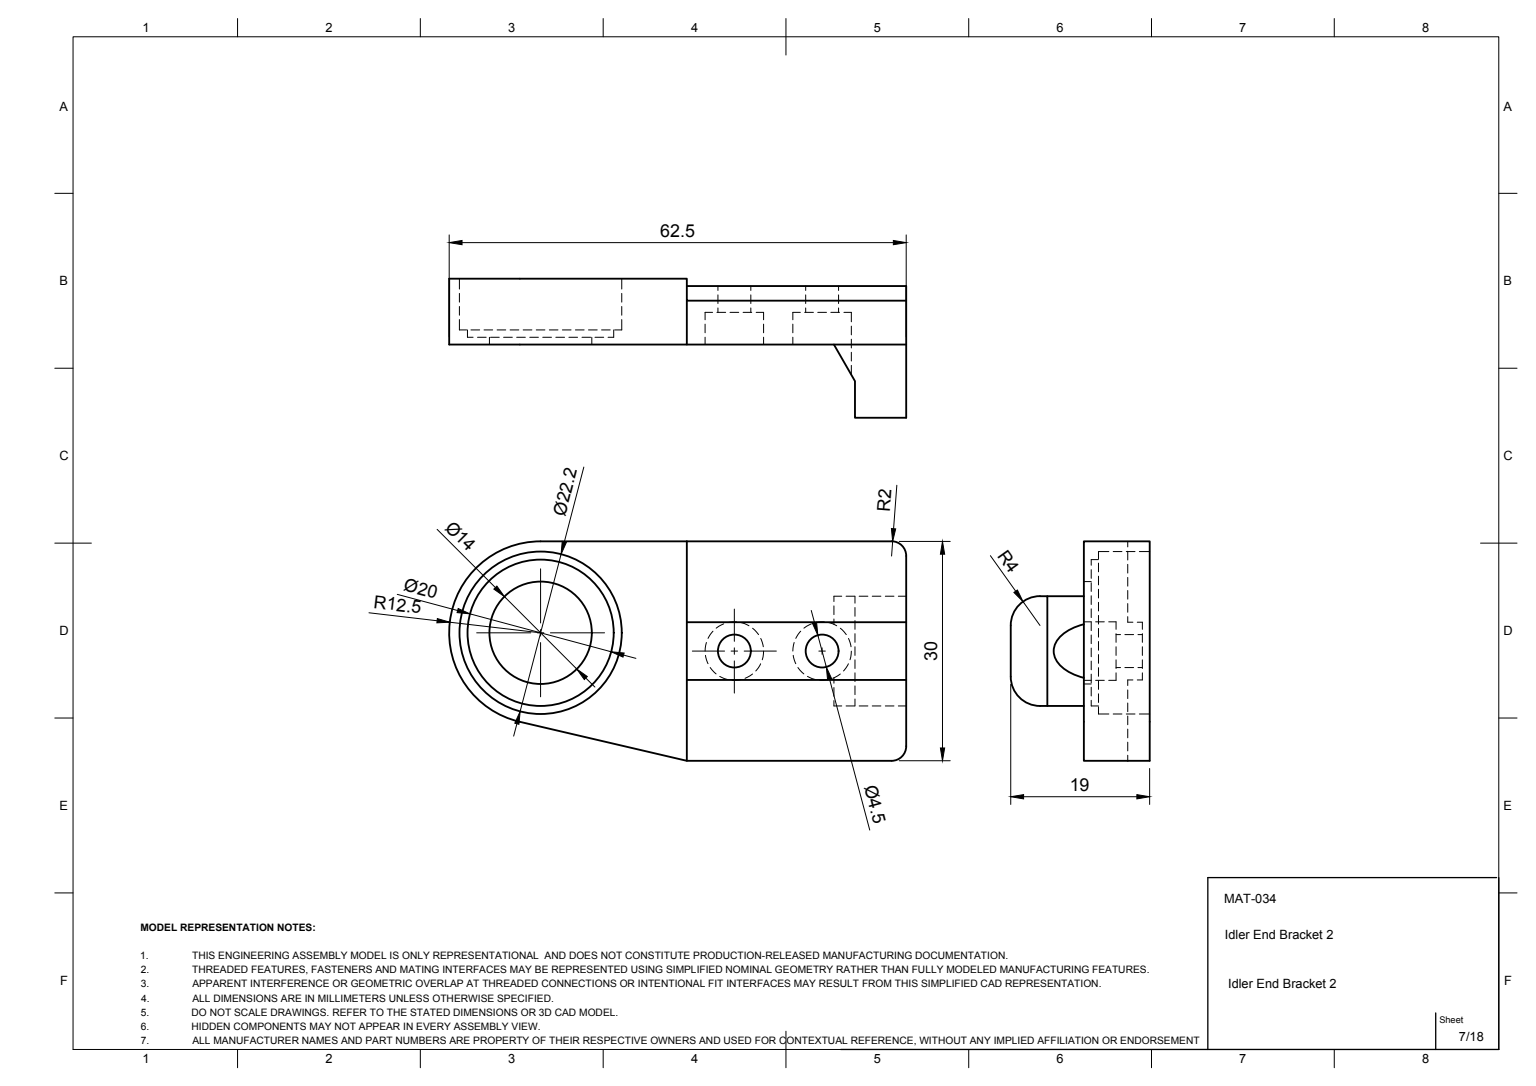
ISO-10303-21;
HEADER;
/* Generated by software containing ST-Developer
 * from STEP Tools, Inc. (www.steptools.com) 
 */

FILE_DESCRIPTION(
/* description */ ('STEP AP214'),
/* implementation_level */ '2;1');

FILE_NAME(
/* name */ 'Idler End Bracket 2.step',
/* time_stamp */ '2026-11-14T09:24:36-08:00',
/* author */ (''),
/* organization */ (''),
/* preprocessor_version */ 'ST-DEVELOPER v20.2',
/* originating_system */ 'Autodesk Translation Framework v15.17.0.0',
/* authorisation */ '');

FILE_SCHEMA (('AUTOMOTIVE_DESIGN { 1 0 10303 214 3 1 1 }'));
ENDSEC;

DATA;
#10=MECHANICAL_DESIGN_GEOMETRIC_PRESENTATION_REPRESENTATION('',(#206),#18867);
#169=ELLIPSE('',#11369,7.99999999999924,3.99999999999989);
#170=ELLIPSE('',#11371,7.99999999999924,3.99999999999989);
#174=SHAPE_REPRESENTATION_RELATIONSHIP('SRR','None',#18938,#190);
#190=ADVANCED_BREP_SHAPE_REPRESENTATION('',(#230),#18854);
#206=STYLED_ITEM('',(#19025),#230);
#230=MANIFOLD_SOLID_BREP('Body1',#10961);
#292=FACE_BOUND('',#1507,.T.);
#293=FACE_BOUND('',#1508,.T.);
#294=FACE_BOUND('',#1510,.T.);
#295=FACE_BOUND('',#1512,.T.);
#296=FACE_BOUND('',#1514,.T.);
#297=FACE_BOUND('',#1518,.T.);
#298=FACE_BOUND('',#1520,.T.);
#299=FACE_BOUND('',#1529,.T.);
#300=FACE_BOUND('',#1530,.T.);
#474=PLANE('',#11390);
#475=PLANE('',#11392);
#476=PLANE('',#11394);
#477=PLANE('',#11395);
#478=PLANE('',#11399);
#479=PLANE('',#11400);
#480=PLANE('',#11403);
#481=PLANE('',#11404);
#482=PLANE('',#11407);
#483=PLANE('',#11408);
#484=PLANE('',#11409);
#485=PLANE('',#11412);
#486=PLANE('',#11413);
#487=PLANE('',#11414);
#488=PLANE('',#11415);
#489=PLANE('',#11418);
#490=PLANE('',#11419);
#491=PLANE('',#11422);
#492=PLANE('',#11423);
#493=PLANE('',#11424);
#494=PLANE('',#11425);
#854=FACE_OUTER_BOUND('',#1491,.T.);
#855=FACE_OUTER_BOUND('',#1492,.T.);
#856=FACE_OUTER_BOUND('',#1493,.T.);
#857=FACE_OUTER_BOUND('',#1494,.T.);
#858=FACE_OUTER_BOUND('',#1495,.T.);
#859=FACE_OUTER_BOUND('',#1496,.T.);
#860=FACE_OUTER_BOUND('',#1497,.T.);
#861=FACE_OUTER_BOUND('',#1498,.T.);
#862=FACE_OUTER_BOUND('',#1499,.T.);
#863=FACE_OUTER_BOUND('',#1500,.T.);
#864=FACE_OUTER_BOUND('',#1501,.T.);
#865=FACE_OUTER_BOUND('',#1502,.T.);
#866=FACE_OUTER_BOUND('',#1503,.T.);
#867=FACE_OUTER_BOUND('',#1504,.T.);
#868=FACE_OUTER_BOUND('',#1505,.T.);
#869=FACE_OUTER_BOUND('',#1506,.T.);
#870=FACE_OUTER_BOUND('',#1509,.T.);
#871=FACE_OUTER_BOUND('',#1511,.T.);
#872=FACE_OUTER_BOUND('',#1513,.T.);
#873=FACE_OUTER_BOUND('',#1515,.T.);
#874=FACE_OUTER_BOUND('',#1516,.T.);
#875=FACE_OUTER_BOUND('',#1517,.T.);
#876=FACE_OUTER_BOUND('',#1519,.T.);
#877=FACE_OUTER_BOUND('',#1521,.T.);
#878=FACE_OUTER_BOUND('',#1522,.T.);
#879=FACE_OUTER_BOUND('',#1523,.T.);
#880=FACE_OUTER_BOUND('',#1524,.T.);
#881=FACE_OUTER_BOUND('',#1525,.T.);
#882=FACE_OUTER_BOUND('',#1526,.T.);
#883=FACE_OUTER_BOUND('',#1527,.T.);
#884=FACE_OUTER_BOUND('',#1528,.T.);
#885=FACE_OUTER_BOUND('',#1531,.T.);
#886=FACE_OUTER_BOUND('',#1532,.T.);
#1491=EDGE_LOOP('',(#7750,#7751,#7752,#7753,#7754,#7755));
#1492=EDGE_LOOP('',(#7756,#7757,#7758,#7759));
#1493=EDGE_LOOP('',(#7760,#7761,#7762,#7763));
#1494=EDGE_LOOP('',(#7764,#7765,#7766,#7767));
#1495=EDGE_LOOP('',(#7768,#7769,#7770,#7771));
#1496=EDGE_LOOP('',(#7772,#7773,#7774,#7775));
#1497=EDGE_LOOP('',(#7776,#7777,#7778,#7779));
#1498=EDGE_LOOP('',(#7780,#7781,#7782,#7783,#7784));
#1499=EDGE_LOOP('',(#7785,#7786,#7787,#7788,#7789));
#1500=EDGE_LOOP('',(#7790,#7791,#7792,#7793,#7794,#7795,#7796,#7797));
#1501=EDGE_LOOP('',(#7798,#7799,#7800,#7801,#7802));
#1502=EDGE_LOOP('',(#7803,#7804,#7805,#7806));
#1503=EDGE_LOOP('',(#7807,#7808,#7809,#7810,#7811,#7812));
#1504=EDGE_LOOP('',(#7813,#7814,#7815,#7816,#7817,#7818,#7819,#7820,#7821,
#7822,#7823,#7824,#7825,#7826));
#1505=EDGE_LOOP('',(#7827,#7828,#7829,#7830));
#1506=EDGE_LOOP('',(#7831,#7832,#7833,#7834,#7835,#7836,#7837,#7838,#7839,
#7840,#7841,#7842,#7843));
#1507=EDGE_LOOP('',(#7844));
#1508=EDGE_LOOP('',(#7845));
#1509=EDGE_LOOP('',(#7846,#7847,#7848,#7849));
#1510=EDGE_LOOP('',(#7850));
#1511=EDGE_LOOP('',(#7851));
#1512=EDGE_LOOP('',(#7852));
#1513=EDGE_LOOP('',(#7853));
#1514=EDGE_LOOP('',(#7854));
#1515=EDGE_LOOP('',(#7855,#7856,#7857,#7858));
#1516=EDGE_LOOP('',(#7859,#7860,#7861,#7862));
#1517=EDGE_LOOP('',(#7863));
#1518=EDGE_LOOP('',(#7864));
#1519=EDGE_LOOP('',(#7865));
#1520=EDGE_LOOP('',(#7866));
#1521=EDGE_LOOP('',(#7867,#7868,#7869,#7870,#7871));
#1522=EDGE_LOOP('',(#7872,#7873,#7874,#7875,#7876,#7877));
#1523=EDGE_LOOP('',(#7878,#7879,#7880,#7881,#7882));
#1524=EDGE_LOOP('',(#7883,#7884,#7885,#7886));
#1525=EDGE_LOOP('',(#7887,#7888,#7889,#7890));
#1526=EDGE_LOOP('',(#7891,#7892,#7893,#7894));
#1527=EDGE_LOOP('',(#7895,#7896,#7897,#7898,#7899,#7900,#7901));
#1528=EDGE_LOOP('',(#7902,#7903,#7904,#7905));
#1529=EDGE_LOOP('',(#7906));
#1530=EDGE_LOOP('',(#7907));
#1531=EDGE_LOOP('',(#7908,#7909,#7910,#7911));
#1532=EDGE_LOOP('',(#7912,#7913,#7914,#7915));
#2294=LINE('',#16277,#3308);
#2295=LINE('',#16287,#3309);
#2296=LINE('',#16293,#3310);
#2297=LINE('',#16299,#3311);
#2298=LINE('',#16305,#3312);
#2299=LINE('',#16311,#3313);
#2300=LINE('',#16317,#3314);
#2301=LINE('',#16322,#3315);
#2302=LINE('',#16324,#3316);
#2303=LINE('',#16328,#3317);
#2304=LINE('',#16329,#3318);
#2305=LINE('',#16333,#3319);
#2306=LINE('',#16335,#3320);
#2307=LINE('',#16337,#3321);
#2308=LINE('',#16340,#3322);
#2309=LINE('',#16343,#3323);
#2310=LINE('',#16345,#3324);
#2311=LINE('',#16347,#3325);
#2312=LINE('',#16348,#3326);
#2313=LINE('',#16350,#3327);
#2314=LINE('',#16351,#3328);
#2315=LINE('',#16354,#3329);
#2316=LINE('',#16356,#3330);
#2317=LINE('',#16358,#3331);
#2318=LINE('',#16359,#3332);
#2319=LINE('',#16364,#3333);
#2320=LINE('',#16368,#3334);
#2321=LINE('',#16369,#3335);
#2322=LINE('',#16370,#3336);
#2323=LINE('',#16373,#3337);
#2324=LINE('',#16375,#3338);
#2325=LINE('',#16377,#3339);
#2326=LINE('',#16378,#3340);
#2327=LINE('',#16380,#3341);
#2328=LINE('',#16382,#3342);
#2329=LINE('',#16384,#3343);
#2330=LINE('',#16388,#3344);
#2331=LINE('',#16392,#3345);
#2332=LINE('',#16393,#3346);
#2333=LINE('',#16396,#3347);
#2334=LINE('',#16397,#3348);
#2335=LINE('',#16400,#3349);
#2336=LINE('',#16401,#3350);
#2337=LINE('',#16403,#3351);
#2338=LINE('',#16404,#3352);
#2339=LINE('',#16417,#3353);
#2340=LINE('',#16418,#3354);
#2341=LINE('',#16419,#3355);
#2342=LINE('',#16422,#3356);
#2343=LINE('',#16424,#3357);
#2344=LINE('',#16428,#3358);
#2345=LINE('',#16431,#3359);
#2346=LINE('',#16432,#3360);
#2347=LINE('',#16434,#3361);
#2348=LINE('',#16435,#3362);
#2349=LINE('',#16440,#3363);
#2350=LINE('',#16441,#3364);
#3308=VECTOR('',#12970,4.);
#3309=VECTOR('',#12981,2.25);
#3310=VECTOR('',#12988,4.);
#3311=VECTOR('',#12995,2.25);
#3312=VECTOR('',#13002,7.00000000000001);
#3313=VECTOR('',#13009,10.);
#3314=VECTOR('',#13016,11.1);
#3315=VECTOR('',#13021,1000.);
#3316=VECTOR('',#13022,1000.);
#3317=VECTOR('',#13025,1000.);
#3318=VECTOR('',#13026,1000.);
#3319=VECTOR('',#13029,1000.);
#3320=VECTOR('',#13030,1000.);
#3321=VECTOR('',#13031,1000.);
#3322=VECTOR('',#13034,1000.);
#3323=VECTOR('',#13037,1000.);
#3324=VECTOR('',#13038,1000.);
#3325=VECTOR('',#13039,1000.);
#3326=VECTOR('',#13040,1000.);
#3327=VECTOR('',#13041,1000.);
#3328=VECTOR('',#13042,1000.);
#3329=VECTOR('',#13045,1000.);
#3330=VECTOR('',#13046,1000.);
#3331=VECTOR('',#13047,1000.);
#3332=VECTOR('',#13048,1000.);
#3333=VECTOR('',#13053,1000.);
#3334=VECTOR('',#13058,1000.);
#3335=VECTOR('',#13059,1000.);
#3336=VECTOR('',#13060,1000.);
#3337=VECTOR('',#13063,1000.);
#3338=VECTOR('',#13064,1000.);
#3339=VECTOR('',#13065,1000.);
#3340=VECTOR('',#13066,1000.);
#3341=VECTOR('',#13067,1000.);
#3342=VECTOR('',#13068,1000.);
#3343=VECTOR('',#13069,1000.);
#3344=VECTOR('',#13072,1000.);
#3345=VECTOR('',#13075,1000.);
#3346=VECTOR('',#13076,1000.);
#3347=VECTOR('',#13079,1000.);
#3348=VECTOR('',#13080,1000.);
#3349=VECTOR('',#13083,1000.);
#3350=VECTOR('',#13084,1000.);
#3351=VECTOR('',#13085,1000.);
#3352=VECTOR('',#13086,1000.);
#3353=VECTOR('',#13107,1000.);
#3354=VECTOR('',#13108,1000.);
#3355=VECTOR('',#13109,1000.);
#3356=VECTOR('',#13112,1000.);
#3357=VECTOR('',#13113,1000.);
#3358=VECTOR('',#13116,1000.);
#3359=VECTOR('',#13121,1000.);
#3360=VECTOR('',#13122,1000.);
#3361=VECTOR('',#13125,1000.);
#3362=VECTOR('',#13126,1000.);
#3363=VECTOR('',#13135,1000.);
#3364=VECTOR('',#13136,1000.);
#4147=CIRCLE('',#11368,4.);
#4148=CIRCLE('',#11370,4.);
#4149=CIRCLE('',#11373,2.25);
#4150=CIRCLE('',#11374,2.25);
#4151=CIRCLE('',#11376,4.);
#4152=CIRCLE('',#11377,4.);
#4153=CIRCLE('',#11379,2.25);
#4154=CIRCLE('',#11380,2.25);
#4155=CIRCLE('',#11382,7.00000000000001);
#4156=CIRCLE('',#11383,7.00000000000001);
#4157=CIRCLE('',#11385,10.);
#4158=CIRCLE('',#11386,10.);
#4159=CIRCLE('',#11388,11.1);
#4160=CIRCLE('',#11389,11.1);
#4161=CIRCLE('',#11391,2.);
#4162=CIRCLE('',#11393,2.);
#4163=CIRCLE('',#11397,12.5);
#4164=CIRCLE('',#11398,12.5);
#4165=CIRCLE('',#11401,4.);
#4166=CIRCLE('',#11402,4.);
#4167=CIRCLE('',#11405,2.);
#4168=CIRCLE('',#11406,2.);
#4169=CIRCLE('',#11416,4.);
#4170=CIRCLE('',#11417,4.);
#4787=VERTEX_POINT('',#16274);
#4788=VERTEX_POINT('',#16276);
#4789=VERTEX_POINT('',#16278);
#4790=VERTEX_POINT('',#16280);
#4791=VERTEX_POINT('',#16284);
#4792=VERTEX_POINT('',#16286);
#4793=VERTEX_POINT('',#16290);
#4794=VERTEX_POINT('',#16292);
#4795=VERTEX_POINT('',#16296);
#4796=VERTEX_POINT('',#16298);
#4797=VERTEX_POINT('',#16302);
#4798=VERTEX_POINT('',#16304);
#4799=VERTEX_POINT('',#16308);
#4800=VERTEX_POINT('',#16310);
#4801=VERTEX_POINT('',#16314);
#4802=VERTEX_POINT('',#16316);
#4803=VERTEX_POINT('',#16320);
#4804=VERTEX_POINT('',#16321);
#4805=VERTEX_POINT('',#16323);
#4806=VERTEX_POINT('',#16325);
#4807=VERTEX_POINT('',#16327);
#4808=VERTEX_POINT('',#16331);
#4809=VERTEX_POINT('',#16332);
#4810=VERTEX_POINT('',#16334);
#4811=VERTEX_POINT('',#16336);
#4812=VERTEX_POINT('',#16338);
#4813=VERTEX_POINT('',#16342);
#4814=VERTEX_POINT('',#16344);
#4815=VERTEX_POINT('',#16346);
#4816=VERTEX_POINT('',#16349);
#4817=VERTEX_POINT('',#16353);
#4818=VERTEX_POINT('',#16355);
#4819=VERTEX_POINT('',#16357);
#4820=VERTEX_POINT('',#16361);
#4821=VERTEX_POINT('',#16363);
#4822=VERTEX_POINT('',#16367);
#4823=VERTEX_POINT('',#16372);
#4824=VERTEX_POINT('',#16374);
#4825=VERTEX_POINT('',#16376);
#4826=VERTEX_POINT('',#16379);
#4827=VERTEX_POINT('',#16381);
#4828=VERTEX_POINT('',#16383);
#4829=VERTEX_POINT('',#16385);
#4830=VERTEX_POINT('',#16387);
#4831=VERTEX_POINT('',#16389);
#4832=VERTEX_POINT('',#16391);
#4833=VERTEX_POINT('',#16395);
#4834=VERTEX_POINT('',#16399);
#4835=VERTEX_POINT('',#16402);
#4836=VERTEX_POINT('',#16415);
#4837=VERTEX_POINT('',#16416);
#4838=VERTEX_POINT('',#16421);
#4839=VERTEX_POINT('',#16423);
#4840=VERTEX_POINT('',#16425);
#4841=VERTEX_POINT('',#16427);
#5908=EDGE_CURVE('',#4787,#4787,#4147,.T.);
#5909=EDGE_CURVE('',#4787,#4788,#2294,.T.);
#5910=EDGE_CURVE('',#4788,#4789,#169,.T.);
#5911=EDGE_CURVE('',#4789,#4790,#4148,.T.);
#5912=EDGE_CURVE('',#4790,#4788,#170,.T.);
#5913=EDGE_CURVE('',#4791,#4791,#4149,.T.);
#5914=EDGE_CURVE('',#4791,#4792,#2295,.T.);
#5915=EDGE_CURVE('',#4792,#4792,#4150,.T.);
#5916=EDGE_CURVE('',#4793,#4793,#4151,.T.);
#5917=EDGE_CURVE('',#4793,#4794,#2296,.T.);
#5918=EDGE_CURVE('',#4794,#4794,#4152,.T.);
#5919=EDGE_CURVE('',#4795,#4795,#4153,.T.);
#5920=EDGE_CURVE('',#4795,#4796,#2297,.T.);
#5921=EDGE_CURVE('',#4796,#4796,#4154,.T.);
#5922=EDGE_CURVE('',#4797,#4797,#4155,.T.);
#5923=EDGE_CURVE('',#4797,#4798,#2298,.T.);
#5924=EDGE_CURVE('',#4798,#4798,#4156,.T.);
#5925=EDGE_CURVE('',#4799,#4799,#4157,.T.);
#5926=EDGE_CURVE('',#4799,#4800,#2299,.T.);
#5927=EDGE_CURVE('',#4800,#4800,#4158,.T.);
#5928=EDGE_CURVE('',#4801,#4801,#4159,.T.);
#5929=EDGE_CURVE('',#4801,#4802,#2300,.T.);
#5930=EDGE_CURVE('',#4802,#4802,#4160,.T.);
#5931=EDGE_CURVE('',#4803,#4804,#2301,.T.);
#5932=EDGE_CURVE('',#4803,#4805,#2302,.T.);
#5933=EDGE_CURVE('',#4805,#4806,#4161,.T.);
#5934=EDGE_CURVE('',#4806,#4807,#2303,.T.);
#5935=EDGE_CURVE('',#4804,#4807,#2304,.T.);
#5936=EDGE_CURVE('',#4808,#4809,#2305,.T.);
#5937=EDGE_CURVE('',#4810,#4808,#2306,.T.);
#5938=EDGE_CURVE('',#4811,#4810,#2307,.T.);
#5939=EDGE_CURVE('',#4811,#4812,#4162,.T.);
#5940=EDGE_CURVE('',#4812,#4809,#2308,.T.);
#5941=EDGE_CURVE('',#4813,#4804,#2309,.T.);
#5942=EDGE_CURVE('',#4807,#4814,#2310,.T.);
#5943=EDGE_CURVE('',#4815,#4814,#2311,.T.);
#5944=EDGE_CURVE('',#4810,#4815,#2312,.T.);
#5945=EDGE_CURVE('',#4816,#4808,#2313,.T.);
#5946=EDGE_CURVE('',#4813,#4816,#2314,.T.);
#5947=EDGE_CURVE('',#4817,#4815,#2315,.T.);
#5948=EDGE_CURVE('',#4818,#4817,#2316,.T.);
#5949=EDGE_CURVE('',#4818,#4819,#2317,.T.);
#5950=EDGE_CURVE('',#4819,#4810,#2318,.T.);
#5951=EDGE_CURVE('',#4817,#4820,#4163,.T.);
#5952=EDGE_CURVE('',#4821,#4820,#2319,.T.);
#5953=EDGE_CURVE('',#4818,#4821,#4164,.T.);
#5954=EDGE_CURVE('',#4806,#4822,#2320,.T.);
#5955=EDGE_CURVE('',#4822,#4821,#2321,.T.);
#5956=EDGE_CURVE('',#4814,#4820,#2322,.T.);
#5957=EDGE_CURVE('',#4823,#4805,#2323,.T.);
#5958=EDGE_CURVE('',#4824,#4803,#2324,.T.);
#5959=EDGE_CURVE('',#4825,#4824,#2325,.T.);
#5960=EDGE_CURVE('',#4825,#4809,#2326,.T.);
#5961=EDGE_CURVE('',#4812,#4826,#2327,.T.);
#5962=EDGE_CURVE('',#4827,#4826,#2328,.T.);
#5963=EDGE_CURVE('',#4828,#4827,#2329,.T.);
#5964=EDGE_CURVE('',#4828,#4829,#4165,.T.);
#5965=EDGE_CURVE('',#4830,#4829,#2330,.T.);
#5966=EDGE_CURVE('',#4830,#4831,#4166,.T.);
#5967=EDGE_CURVE('',#4831,#4832,#2331,.T.);
#5968=EDGE_CURVE('',#4823,#4832,#2332,.T.);
#5969=EDGE_CURVE('',#4833,#4811,#2333,.T.);
#5970=EDGE_CURVE('',#4833,#4819,#2334,.T.);
#5971=EDGE_CURVE('',#4834,#4832,#2335,.T.);
#5972=EDGE_CURVE('',#4834,#4790,#2336,.T.);
#5973=EDGE_CURVE('',#4789,#4835,#2337,.T.);
#5974=EDGE_CURVE('',#4827,#4835,#2338,.T.);
#5975=EDGE_CURVE('',#4826,#4833,#4167,.T.);
#5976=EDGE_CURVE('',#4822,#4823,#4168,.T.);
#5977=EDGE_CURVE('',#4836,#4837,#2339,.T.);
#5978=EDGE_CURVE('',#4836,#4828,#2340,.T.);
#5979=EDGE_CURVE('',#4835,#4837,#2341,.T.);
#5980=EDGE_CURVE('',#4837,#4838,#2342,.T.);
#5981=EDGE_CURVE('',#4839,#4838,#2343,.T.);
#5982=EDGE_CURVE('',#4839,#4840,#4169,.T.);
#5983=EDGE_CURVE('',#4841,#4840,#2344,.T.);
#5984=EDGE_CURVE('',#4841,#4836,#4170,.T.);
#5985=EDGE_CURVE('',#4831,#4839,#2345,.T.);
#5986=EDGE_CURVE('',#4838,#4834,#2346,.T.);
#5987=EDGE_CURVE('',#4840,#4830,#2347,.T.);
#5988=EDGE_CURVE('',#4829,#4841,#2348,.T.);
#5989=EDGE_CURVE('',#4824,#4813,#2349,.T.);
#5990=EDGE_CURVE('',#4816,#4825,#2350,.T.);
#7750=ORIENTED_EDGE('',*,*,#5908,.F.);
#7751=ORIENTED_EDGE('',*,*,#5909,.T.);
#7752=ORIENTED_EDGE('',*,*,#5910,.T.);
#7753=ORIENTED_EDGE('',*,*,#5911,.T.);
#7754=ORIENTED_EDGE('',*,*,#5912,.T.);
#7755=ORIENTED_EDGE('',*,*,#5909,.F.);
#7756=ORIENTED_EDGE('',*,*,#5913,.T.);
#7757=ORIENTED_EDGE('',*,*,#5914,.T.);
#7758=ORIENTED_EDGE('',*,*,#5915,.T.);
#7759=ORIENTED_EDGE('',*,*,#5914,.F.);
#7760=ORIENTED_EDGE('',*,*,#5916,.F.);
#7761=ORIENTED_EDGE('',*,*,#5917,.T.);
#7762=ORIENTED_EDGE('',*,*,#5918,.T.);
#7763=ORIENTED_EDGE('',*,*,#5917,.F.);
#7764=ORIENTED_EDGE('',*,*,#5919,.T.);
#7765=ORIENTED_EDGE('',*,*,#5920,.T.);
#7766=ORIENTED_EDGE('',*,*,#5921,.T.);
#7767=ORIENTED_EDGE('',*,*,#5920,.F.);
#7768=ORIENTED_EDGE('',*,*,#5922,.F.);
#7769=ORIENTED_EDGE('',*,*,#5923,.T.);
#7770=ORIENTED_EDGE('',*,*,#5924,.T.);
#7771=ORIENTED_EDGE('',*,*,#5923,.F.);
#7772=ORIENTED_EDGE('',*,*,#5925,.F.);
#7773=ORIENTED_EDGE('',*,*,#5926,.T.);
#7774=ORIENTED_EDGE('',*,*,#5927,.T.);
#7775=ORIENTED_EDGE('',*,*,#5926,.F.);
#7776=ORIENTED_EDGE('',*,*,#5928,.F.);
#7777=ORIENTED_EDGE('',*,*,#5929,.T.);
#7778=ORIENTED_EDGE('',*,*,#5930,.T.);
#7779=ORIENTED_EDGE('',*,*,#5929,.F.);
#7780=ORIENTED_EDGE('',*,*,#5931,.F.);
#7781=ORIENTED_EDGE('',*,*,#5932,.T.);
#7782=ORIENTED_EDGE('',*,*,#5933,.T.);
#7783=ORIENTED_EDGE('',*,*,#5934,.T.);
#7784=ORIENTED_EDGE('',*,*,#5935,.F.);
#7785=ORIENTED_EDGE('',*,*,#5936,.F.);
#7786=ORIENTED_EDGE('',*,*,#5937,.F.);
#7787=ORIENTED_EDGE('',*,*,#5938,.F.);
#7788=ORIENTED_EDGE('',*,*,#5939,.T.);
#7789=ORIENTED_EDGE('',*,*,#5940,.T.);
#7790=ORIENTED_EDGE('',*,*,#5941,.T.);
#7791=ORIENTED_EDGE('',*,*,#5935,.T.);
#7792=ORIENTED_EDGE('',*,*,#5942,.T.);
#7793=ORIENTED_EDGE('',*,*,#5943,.F.);
#7794=ORIENTED_EDGE('',*,*,#5944,.F.);
#7795=ORIENTED_EDGE('',*,*,#5937,.T.);
#7796=ORIENTED_EDGE('',*,*,#5945,.F.);
#7797=ORIENTED_EDGE('',*,*,#5946,.F.);
#7798=ORIENTED_EDGE('',*,*,#5947,.F.);
#7799=ORIENTED_EDGE('',*,*,#5948,.F.);
#7800=ORIENTED_EDGE('',*,*,#5949,.T.);
#7801=ORIENTED_EDGE('',*,*,#5950,.T.);
#7802=ORIENTED_EDGE('',*,*,#5944,.T.);
#7803=ORIENTED_EDGE('',*,*,#5951,.T.);
#7804=ORIENTED_EDGE('',*,*,#5952,.F.);
#7805=ORIENTED_EDGE('',*,*,#5953,.F.);
#7806=ORIENTED_EDGE('',*,*,#5948,.T.);
#7807=ORIENTED_EDGE('',*,*,#5942,.F.);
#7808=ORIENTED_EDGE('',*,*,#5934,.F.);
#7809=ORIENTED_EDGE('',*,*,#5954,.T.);
#7810=ORIENTED_EDGE('',*,*,#5955,.T.);
#7811=ORIENTED_EDGE('',*,*,#5952,.T.);
#7812=ORIENTED_EDGE('',*,*,#5956,.F.);
#7813=ORIENTED_EDGE('',*,*,#5957,.T.);
#7814=ORIENTED_EDGE('',*,*,#5932,.F.);
#7815=ORIENTED_EDGE('',*,*,#5958,.F.);
#7816=ORIENTED_EDGE('',*,*,#5959,.F.);
#7817=ORIENTED_EDGE('',*,*,#5960,.T.);
#7818=ORIENTED_EDGE('',*,*,#5940,.F.);
#7819=ORIENTED_EDGE('',*,*,#5961,.T.);
#7820=ORIENTED_EDGE('',*,*,#5962,.F.);
#7821=ORIENTED_EDGE('',*,*,#5963,.F.);
#7822=ORIENTED_EDGE('',*,*,#5964,.T.);
#7823=ORIENTED_EDGE('',*,*,#5965,.F.);
#7824=ORIENTED_EDGE('',*,*,#5966,.T.);
#7825=ORIENTED_EDGE('',*,*,#5967,.T.);
#7826=ORIENTED_EDGE('',*,*,#5968,.F.);
#7827=ORIENTED_EDGE('',*,*,#5969,.T.);
#7828=ORIENTED_EDGE('',*,*,#5938,.T.);
#7829=ORIENTED_EDGE('',*,*,#5950,.F.);
#7830=ORIENTED_EDGE('',*,*,#5970,.F.);
#7831=ORIENTED_EDGE('',*,*,#5971,.F.);
#7832=ORIENTED_EDGE('',*,*,#5972,.T.);
#7833=ORIENTED_EDGE('',*,*,#5911,.F.);
#7834=ORIENTED_EDGE('',*,*,#5973,.T.);
#7835=ORIENTED_EDGE('',*,*,#5974,.F.);
#7836=ORIENTED_EDGE('',*,*,#5962,.T.);
#7837=ORIENTED_EDGE('',*,*,#5975,.T.);
#7838=ORIENTED_EDGE('',*,*,#5970,.T.);
#7839=ORIENTED_EDGE('',*,*,#5949,.F.);
#7840=ORIENTED_EDGE('',*,*,#5953,.T.);
#7841=ORIENTED_EDGE('',*,*,#5955,.F.);
#7842=ORIENTED_EDGE('',*,*,#5976,.T.);
#7843=ORIENTED_EDGE('',*,*,#5968,.T.);
#7844=ORIENTED_EDGE('',*,*,#5918,.F.);
#7845=ORIENTED_EDGE('',*,*,#5922,.T.);
#7846=ORIENTED_EDGE('',*,*,#5947,.T.);
#7847=ORIENTED_EDGE('',*,*,#5943,.T.);
#7848=ORIENTED_EDGE('',*,*,#5956,.T.);
#7849=ORIENTED_EDGE('',*,*,#5951,.F.);
#7850=ORIENTED_EDGE('',*,*,#5930,.F.);
#7851=ORIENTED_EDGE('',*,*,#5928,.T.);
#7852=ORIENTED_EDGE('',*,*,#5927,.F.);
#7853=ORIENTED_EDGE('',*,*,#5925,.T.);
#7854=ORIENTED_EDGE('',*,*,#5924,.F.);
#7855=ORIENTED_EDGE('',*,*,#5939,.F.);
#7856=ORIENTED_EDGE('',*,*,#5969,.F.);
#7857=ORIENTED_EDGE('',*,*,#5975,.F.);
#7858=ORIENTED_EDGE('',*,*,#5961,.F.);
#7859=ORIENTED_EDGE('',*,*,#5933,.F.);
#7860=ORIENTED_EDGE('',*,*,#5957,.F.);
#7861=ORIENTED_EDGE('',*,*,#5976,.F.);
#7862=ORIENTED_EDGE('',*,*,#5954,.F.);
#7863=ORIENTED_EDGE('',*,*,#5916,.T.);
#7864=ORIENTED_EDGE('',*,*,#5921,.F.);
#7865=ORIENTED_EDGE('',*,*,#5908,.T.);
#7866=ORIENTED_EDGE('',*,*,#5915,.F.);
#7867=ORIENTED_EDGE('',*,*,#5977,.F.);
#7868=ORIENTED_EDGE('',*,*,#5978,.T.);
#7869=ORIENTED_EDGE('',*,*,#5963,.T.);
#7870=ORIENTED_EDGE('',*,*,#5974,.T.);
#7871=ORIENTED_EDGE('',*,*,#5979,.T.);
#7872=ORIENTED_EDGE('',*,*,#5977,.T.);
#7873=ORIENTED_EDGE('',*,*,#5980,.T.);
#7874=ORIENTED_EDGE('',*,*,#5981,.F.);
#7875=ORIENTED_EDGE('',*,*,#5982,.T.);
#7876=ORIENTED_EDGE('',*,*,#5983,.F.);
#7877=ORIENTED_EDGE('',*,*,#5984,.T.);
#7878=ORIENTED_EDGE('',*,*,#5967,.F.);
#7879=ORIENTED_EDGE('',*,*,#5985,.T.);
#7880=ORIENTED_EDGE('',*,*,#5981,.T.);
#7881=ORIENTED_EDGE('',*,*,#5986,.T.);
#7882=ORIENTED_EDGE('',*,*,#5971,.T.);
#7883=ORIENTED_EDGE('',*,*,#5983,.T.);
#7884=ORIENTED_EDGE('',*,*,#5987,.T.);
#7885=ORIENTED_EDGE('',*,*,#5965,.T.);
#7886=ORIENTED_EDGE('',*,*,#5988,.T.);
#7887=ORIENTED_EDGE('',*,*,#5982,.F.);
#7888=ORIENTED_EDGE('',*,*,#5985,.F.);
#7889=ORIENTED_EDGE('',*,*,#5966,.F.);
#7890=ORIENTED_EDGE('',*,*,#5987,.F.);
#7891=ORIENTED_EDGE('',*,*,#5964,.F.);
#7892=ORIENTED_EDGE('',*,*,#5978,.F.);
#7893=ORIENTED_EDGE('',*,*,#5984,.F.);
#7894=ORIENTED_EDGE('',*,*,#5988,.F.);
#7895=ORIENTED_EDGE('',*,*,#5912,.F.);
#7896=ORIENTED_EDGE('',*,*,#5972,.F.);
#7897=ORIENTED_EDGE('',*,*,#5986,.F.);
#7898=ORIENTED_EDGE('',*,*,#5980,.F.);
#7899=ORIENTED_EDGE('',*,*,#5979,.F.);
#7900=ORIENTED_EDGE('',*,*,#5973,.F.);
#7901=ORIENTED_EDGE('',*,*,#5910,.F.);
#7902=ORIENTED_EDGE('',*,*,#5959,.T.);
#7903=ORIENTED_EDGE('',*,*,#5989,.T.);
#7904=ORIENTED_EDGE('',*,*,#5946,.T.);
#7905=ORIENTED_EDGE('',*,*,#5990,.T.);
#7906=ORIENTED_EDGE('',*,*,#5913,.F.);
#7907=ORIENTED_EDGE('',*,*,#5919,.F.);
#7908=ORIENTED_EDGE('',*,*,#5931,.T.);
#7909=ORIENTED_EDGE('',*,*,#5941,.F.);
#7910=ORIENTED_EDGE('',*,*,#5989,.F.);
#7911=ORIENTED_EDGE('',*,*,#5958,.T.);
#7912=ORIENTED_EDGE('',*,*,#5936,.T.);
#7913=ORIENTED_EDGE('',*,*,#5960,.F.);
#7914=ORIENTED_EDGE('',*,*,#5990,.F.);
#7915=ORIENTED_EDGE('',*,*,#5945,.T.);
#10186=CYLINDRICAL_SURFACE('',#11367,4.);
#10187=CYLINDRICAL_SURFACE('',#11372,2.25);
#10188=CYLINDRICAL_SURFACE('',#11375,4.);
#10189=CYLINDRICAL_SURFACE('',#11378,2.25);
#10190=CYLINDRICAL_SURFACE('',#11381,7.00000000000001);
#10191=CYLINDRICAL_SURFACE('',#11384,10.);
#10192=CYLINDRICAL_SURFACE('',#11387,11.1);
#10193=CYLINDRICAL_SURFACE('',#11396,12.5);
#10194=CYLINDRICAL_SURFACE('',#11410,2.);
#10195=CYLINDRICAL_SURFACE('',#11411,2.);
#10196=CYLINDRICAL_SURFACE('',#11420,4.);
#10197=CYLINDRICAL_SURFACE('',#11421,4.);
#10491=ADVANCED_FACE('',(#854),#10186,.F.);
#10492=ADVANCED_FACE('',(#855),#10187,.F.);
#10493=ADVANCED_FACE('',(#856),#10188,.F.);
#10494=ADVANCED_FACE('',(#857),#10189,.F.);
#10495=ADVANCED_FACE('',(#858),#10190,.F.);
#10496=ADVANCED_FACE('',(#859),#10191,.F.);
#10497=ADVANCED_FACE('',(#860),#10192,.F.);
#10498=ADVANCED_FACE('',(#861),#474,.F.);
#10499=ADVANCED_FACE('',(#862),#475,.F.);
#10500=ADVANCED_FACE('',(#863),#476,.F.);
#10501=ADVANCED_FACE('',(#864),#477,.T.);
#10502=ADVANCED_FACE('',(#865),#10193,.T.);
#10503=ADVANCED_FACE('',(#866),#478,.T.);
#10504=ADVANCED_FACE('',(#867),#479,.F.);
#10505=ADVANCED_FACE('',(#868),#480,.F.);
#10506=ADVANCED_FACE('',(#869,#292,#293),#481,.T.);
#10507=ADVANCED_FACE('',(#870,#294),#482,.F.);
#10508=ADVANCED_FACE('',(#871,#295),#483,.T.);
#10509=ADVANCED_FACE('',(#872,#296),#484,.T.);
#10510=ADVANCED_FACE('',(#873),#10194,.T.);
#10511=ADVANCED_FACE('',(#874),#10195,.T.);
#10512=ADVANCED_FACE('',(#875,#297),#485,.F.);
#10513=ADVANCED_FACE('',(#876,#298),#486,.F.);
#10514=ADVANCED_FACE('',(#877),#487,.F.);
#10515=ADVANCED_FACE('',(#878),#488,.F.);
#10516=ADVANCED_FACE('',(#879),#489,.F.);
#10517=ADVANCED_FACE('',(#880),#490,.T.);
#10518=ADVANCED_FACE('',(#881),#10196,.T.);
#10519=ADVANCED_FACE('',(#882),#10197,.T.);
#10520=ADVANCED_FACE('',(#883),#491,.F.);
#10521=ADVANCED_FACE('',(#884,#299,#300),#492,.F.);
#10522=ADVANCED_FACE('',(#885),#493,.F.);
#10523=ADVANCED_FACE('',(#886),#494,.F.);
#10961=CLOSED_SHELL('',(#10491,#10492,#10493,#10494,#10495,#10496,#10497,
#10498,#10499,#10500,#10501,#10502,#10503,#10504,#10505,#10506,#10507,#10508,
#10509,#10510,#10511,#10512,#10513,#10514,#10515,#10516,#10517,#10518,#10519,
#10520,#10521,#10522,#10523));
#11366=AXIS2_PLACEMENT_3D('',#16272,#12964,#12965);
#11367=AXIS2_PLACEMENT_3D('',#16273,#12966,#12967);
#11368=AXIS2_PLACEMENT_3D('',#16275,#12968,#12969);
#11369=AXIS2_PLACEMENT_3D('',#16279,#12971,#12972);
#11370=AXIS2_PLACEMENT_3D('',#16281,#12973,#12974);
#11371=AXIS2_PLACEMENT_3D('',#16282,#12975,#12976);
#11372=AXIS2_PLACEMENT_3D('',#16283,#12977,#12978);
#11373=AXIS2_PLACEMENT_3D('',#16285,#12979,#12980);
#11374=AXIS2_PLACEMENT_3D('',#16288,#12982,#12983);
#11375=AXIS2_PLACEMENT_3D('',#16289,#12984,#12985);
#11376=AXIS2_PLACEMENT_3D('',#16291,#12986,#12987);
#11377=AXIS2_PLACEMENT_3D('',#16294,#12989,#12990);
#11378=AXIS2_PLACEMENT_3D('',#16295,#12991,#12992);
#11379=AXIS2_PLACEMENT_3D('',#16297,#12993,#12994);
#11380=AXIS2_PLACEMENT_3D('',#16300,#12996,#12997);
#11381=AXIS2_PLACEMENT_3D('',#16301,#12998,#12999);
#11382=AXIS2_PLACEMENT_3D('',#16303,#13000,#13001);
#11383=AXIS2_PLACEMENT_3D('',#16306,#13003,#13004);
#11384=AXIS2_PLACEMENT_3D('',#16307,#13005,#13006);
#11385=AXIS2_PLACEMENT_3D('',#16309,#13007,#13008);
#11386=AXIS2_PLACEMENT_3D('',#16312,#13010,#13011);
#11387=AXIS2_PLACEMENT_3D('',#16313,#13012,#13013);
#11388=AXIS2_PLACEMENT_3D('',#16315,#13014,#13015);
#11389=AXIS2_PLACEMENT_3D('',#16318,#13017,#13018);
#11390=AXIS2_PLACEMENT_3D('',#16319,#13019,#13020);
#11391=AXIS2_PLACEMENT_3D('',#16326,#13023,#13024);
#11392=AXIS2_PLACEMENT_3D('',#16330,#13027,#13028);
#11393=AXIS2_PLACEMENT_3D('',#16339,#13032,#13033);
#11394=AXIS2_PLACEMENT_3D('',#16341,#13035,#13036);
#11395=AXIS2_PLACEMENT_3D('',#16352,#13043,#13044);
#11396=AXIS2_PLACEMENT_3D('',#16360,#13049,#13050);
#11397=AXIS2_PLACEMENT_3D('',#16362,#13051,#13052);
#11398=AXIS2_PLACEMENT_3D('',#16365,#13054,#13055);
#11399=AXIS2_PLACEMENT_3D('',#16366,#13056,#13057);
#11400=AXIS2_PLACEMENT_3D('',#16371,#13061,#13062);
#11401=AXIS2_PLACEMENT_3D('',#16386,#13070,#13071);
#11402=AXIS2_PLACEMENT_3D('',#16390,#13073,#13074);
#11403=AXIS2_PLACEMENT_3D('',#16394,#13077,#13078);
#11404=AXIS2_PLACEMENT_3D('',#16398,#13081,#13082);
#11405=AXIS2_PLACEMENT_3D('',#16405,#13087,#13088);
#11406=AXIS2_PLACEMENT_3D('',#16406,#13089,#13090);
#11407=AXIS2_PLACEMENT_3D('',#16407,#13091,#13092);
#11408=AXIS2_PLACEMENT_3D('',#16408,#13093,#13094);
#11409=AXIS2_PLACEMENT_3D('',#16409,#13095,#13096);
#11410=AXIS2_PLACEMENT_3D('',#16410,#13097,#13098);
#11411=AXIS2_PLACEMENT_3D('',#16411,#13099,#13100);
#11412=AXIS2_PLACEMENT_3D('',#16412,#13101,#13102);
#11413=AXIS2_PLACEMENT_3D('',#16413,#13103,#13104);
#11414=AXIS2_PLACEMENT_3D('',#16414,#13105,#13106);
#11415=AXIS2_PLACEMENT_3D('',#16420,#13110,#13111);
#11416=AXIS2_PLACEMENT_3D('',#16426,#13114,#13115);
#11417=AXIS2_PLACEMENT_3D('',#16429,#13117,#13118);
#11418=AXIS2_PLACEMENT_3D('',#16430,#13119,#13120);
#11419=AXIS2_PLACEMENT_3D('',#16433,#13123,#13124);
#11420=AXIS2_PLACEMENT_3D('',#16436,#13127,#13128);
#11421=AXIS2_PLACEMENT_3D('',#16437,#13129,#13130);
#11422=AXIS2_PLACEMENT_3D('',#16438,#13131,#13132);
#11423=AXIS2_PLACEMENT_3D('',#16439,#13133,#13134);
#11424=AXIS2_PLACEMENT_3D('',#16442,#13137,#13138);
#11425=AXIS2_PLACEMENT_3D('',#16443,#13139,#13140);
#12964=DIRECTION('axis',(0.,0.,1.));
#12965=DIRECTION('refdir',(1.,0.,0.));
#12966=DIRECTION('center_axis',(0.,0.,1.));
#12967=DIRECTION('ref_axis',(1.,0.,0.));
#12968=DIRECTION('center_axis',(0.,0.,1.));
#12969=DIRECTION('ref_axis',(1.,0.,0.));
#12970=DIRECTION('',(0.,0.,1.));
#12971=DIRECTION('center_axis',(0.866025403784445,2.62556109623269E-14,
0.499999999999989));
#12972=DIRECTION('ref_axis',(0.499999999999989,-1.95567765134161E-14,-0.866025403784445));
#12973=DIRECTION('center_axis',(0.,0.,1.));
#12974=DIRECTION('ref_axis',(1.,0.,0.));
#12975=DIRECTION('center_axis',(0.866025403784445,2.62556109623269E-14,
0.499999999999989));
#12976=DIRECTION('ref_axis',(0.499999999999989,-1.95567765134161E-14,-0.866025403784445));
#12977=DIRECTION('center_axis',(0.,0.,1.));
#12978=DIRECTION('ref_axis',(1.,0.,0.));
#12979=DIRECTION('center_axis',(0.,0.,-1.));
#12980=DIRECTION('ref_axis',(-1.,0.,0.));
#12981=DIRECTION('',(0.,0.,1.));
#12982=DIRECTION('center_axis',(0.,0.,1.));
#12983=DIRECTION('ref_axis',(1.,0.,0.));
#12984=DIRECTION('center_axis',(0.,0.,1.));
#12985=DIRECTION('ref_axis',(1.,0.,0.));
#12986=DIRECTION('center_axis',(0.,0.,1.));
#12987=DIRECTION('ref_axis',(1.,0.,0.));
#12988=DIRECTION('',(0.,0.,1.));
#12989=DIRECTION('center_axis',(0.,0.,1.));
#12990=DIRECTION('ref_axis',(1.,0.,0.));
#12991=DIRECTION('center_axis',(0.,0.,1.));
#12992=DIRECTION('ref_axis',(1.,0.,0.));
#12993=DIRECTION('center_axis',(0.,0.,-1.));
#12994=DIRECTION('ref_axis',(-1.,0.,0.));
#12995=DIRECTION('',(0.,0.,1.));
#12996=DIRECTION('center_axis',(0.,0.,1.));
#12997=DIRECTION('ref_axis',(1.,0.,0.));
#12998=DIRECTION('center_axis',(0.,0.,-1.));
#12999=DIRECTION('ref_axis',(-1.,0.,0.));
#13000=DIRECTION('center_axis',(0.,0.,-1.));
#13001=DIRECTION('ref_axis',(-1.,0.,0.));
#13002=DIRECTION('',(0.,0.,-1.));
#13003=DIRECTION('center_axis',(0.,0.,-1.));
#13004=DIRECTION('ref_axis',(-1.,0.,0.));
#13005=DIRECTION('center_axis',(0.,0.,-1.));
#13006=DIRECTION('ref_axis',(-1.,0.,0.));
#13007=DIRECTION('center_axis',(0.,0.,-1.));
#13008=DIRECTION('ref_axis',(-1.,0.,0.));
#13009=DIRECTION('',(0.,0.,-1.));
#13010=DIRECTION('center_axis',(0.,0.,-1.));
#13011=DIRECTION('ref_axis',(-1.,0.,0.));
#13012=DIRECTION('center_axis',(0.,0.,-1.));
#13013=DIRECTION('ref_axis',(-1.,0.,0.));
#13014=DIRECTION('center_axis',(0.,0.,-1.));
#13015=DIRECTION('ref_axis',(-1.,0.,0.));
#13016=DIRECTION('',(0.,0.,-1.));
#13017=DIRECTION('center_axis',(0.,0.,-1.));
#13018=DIRECTION('ref_axis',(-1.,0.,0.));
#13019=DIRECTION('center_axis',(0.,0.,1.));
#13020=DIRECTION('ref_axis',(1.,0.,0.));
#13021=DIRECTION('',(1.,0.,0.));
#13022=DIRECTION('',(0.,1.,0.));
#13023=DIRECTION('center_axis',(0.,0.,-1.));
#13024=DIRECTION('ref_axis',(1.,0.,0.));
#13025=DIRECTION('',(1.,0.,0.));
#13026=DIRECTION('',(0.,1.,0.));
#13027=DIRECTION('center_axis',(0.,0.,1.));
#13028=DIRECTION('ref_axis',(1.,0.,0.));
#13029=DIRECTION('',(-1.,-2.89120579329468E-17,0.));
#13030=DIRECTION('',(0.,1.,0.));
#13031=DIRECTION('',(1.,0.,0.));
#13032=DIRECTION('center_axis',(0.,0.,-1.));
#13033=DIRECTION('ref_axis',(1.,0.,0.));
#13034=DIRECTION('',(0.,1.,0.));
#13035=DIRECTION('center_axis',(1.,0.,0.));
#13036=DIRECTION('ref_axis',(0.,0.,-1.));
#13037=DIRECTION('',(0.,0.,1.));
#13038=DIRECTION('',(0.,0.,-1.));
#13039=DIRECTION('',(0.,1.,0.));
#13040=DIRECTION('',(0.,0.,-1.));
#13041=DIRECTION('',(0.,0.,1.));
#13042=DIRECTION('',(0.,-1.,0.));
#13043=DIRECTION('center_axis',(0.227131156084319,-0.973864178382079,0.));
#13044=DIRECTION('ref_axis',(0.973864178382079,0.227131156084319,0.));
#13045=DIRECTION('',(-0.973864178382078,-0.227131156084319,0.));
#13046=DIRECTION('',(0.,0.,-1.));
#13047=DIRECTION('',(-0.973864178382078,-0.227131156084319,0.));
#13048=DIRECTION('',(0.,0.,-1.));
#13049=DIRECTION('center_axis',(0.,0.,-1.));
#13050=DIRECTION('ref_axis',(0.993444557683537,0.114314963189256,0.));
#13051=DIRECTION('center_axis',(0.,0.,1.));
#13052=DIRECTION('ref_axis',(1.,0.,0.));
#13053=DIRECTION('',(0.,0.,-1.));
#13054=DIRECTION('center_axis',(0.,0.,1.));
#13055=DIRECTION('ref_axis',(1.,0.,0.));
#13056=DIRECTION('center_axis',(0.,1.,0.));
#13057=DIRECTION('ref_axis',(0.,0.,1.));
#13058=DIRECTION('',(0.,0.,1.));
#13059=DIRECTION('',(1.,0.,0.));
#13060=DIRECTION('',(1.,0.,0.));
#13061=DIRECTION('center_axis',(1.,0.,0.));
#13062=DIRECTION('ref_axis',(0.,0.,-1.));
#13063=DIRECTION('',(0.,0.,-1.));
#13064=DIRECTION('',(0.,0.,1.));
#13065=DIRECTION('',(0.,1.,0.));
#13066=DIRECTION('',(0.,0.,1.));
#13067=DIRECTION('',(0.,0.,1.));
#13068=DIRECTION('',(0.,-1.,0.));
#13069=DIRECTION('',(0.,0.,-1.));
#13070=DIRECTION('center_axis',(-1.,0.,0.));
#13071=DIRECTION('ref_axis',(0.,0.,-1.));
#13072=DIRECTION('',(0.,-1.,0.));
#13073=DIRECTION('center_axis',(-1.,0.,0.));
#13074=DIRECTION('ref_axis',(0.,0.,-1.));
#13075=DIRECTION('',(0.,0.,-1.));
#13076=DIRECTION('',(0.,-1.,0.));
#13077=DIRECTION('center_axis',(-1.15648231731787E-16,1.,0.));
#13078=DIRECTION('ref_axis',(-1.,-1.15648231731787E-16,0.));
#13079=DIRECTION('',(0.,0.,-1.));
#13080=DIRECTION('',(1.,1.15648231731787E-16,0.));
#13081=DIRECTION('center_axis',(0.,0.,1.));
#13082=DIRECTION('ref_axis',(1.,0.,0.));
#13083=DIRECTION('',(-1.,-1.23908819712629E-16,0.));
#13084=DIRECTION('',(0.,-1.,0.));
#13085=DIRECTION('',(0.,-1.,0.));
#13086=DIRECTION('',(1.,1.23908819712629E-16,0.));
#13087=DIRECTION('center_axis',(0.,0.,1.));
#13088=DIRECTION('ref_axis',(1.,0.,0.));
#13089=DIRECTION('center_axis',(0.,0.,1.));
#13090=DIRECTION('ref_axis',(1.,0.,0.));
#13091=DIRECTION('center_axis',(0.,0.,1.));
#13092=DIRECTION('ref_axis',(1.,0.,0.));
#13093=DIRECTION('center_axis',(0.,0.,-1.));
#13094=DIRECTION('ref_axis',(-1.,0.,0.));
#13095=DIRECTION('center_axis',(0.,0.,-1.));
#13096=DIRECTION('ref_axis',(-1.,0.,0.));
#13097=DIRECTION('center_axis',(0.,0.,-1.));
#13098=DIRECTION('ref_axis',(-1.,0.,0.));
#13099=DIRECTION('center_axis',(0.,0.,1.));
#13100=DIRECTION('ref_axis',(1.,0.,0.));
#13101=DIRECTION('center_axis',(0.,0.,-1.));
#13102=DIRECTION('ref_axis',(-1.,0.,0.));
#13103=DIRECTION('center_axis',(0.,0.,-1.));
#13104=DIRECTION('ref_axis',(-1.,0.,0.));
#13105=DIRECTION('center_axis',(-1.23908819712629E-16,1.,0.));
#13106=DIRECTION('ref_axis',(-1.,-1.23908819712629E-16,0.));
#13107=DIRECTION('',(0.,0.,-1.));
#13108=DIRECTION('',(-1.,-1.23908819712629E-16,0.));
#13109=DIRECTION('',(-0.500000000000005,-6.19544098563151E-17,0.866025403784436));
#13110=DIRECTION('center_axis',(-1.,0.,0.));
#13111=DIRECTION('ref_axis',(0.,0.,1.));
#13112=DIRECTION('',(0.,1.,0.));
#13113=DIRECTION('',(0.,0.,-1.));
#13114=DIRECTION('center_axis',(1.,0.,0.));
#13115=DIRECTION('ref_axis',(0.,0.,1.));
#13116=DIRECTION('',(0.,1.,0.));
#13117=DIRECTION('center_axis',(1.,0.,0.));
#13118=DIRECTION('ref_axis',(0.,0.,1.));
#13119=DIRECTION('center_axis',(1.23908819712629E-16,-1.,0.));
#13120=DIRECTION('ref_axis',(1.,1.23908819712629E-16,0.));
#13121=DIRECTION('',(1.,1.23908819712629E-16,0.));
#13122=DIRECTION('',(0.500000000000005,6.19544098563151E-17,-0.866025403784436));
#13123=DIRECTION('center_axis',(0.,0.,1.));
#13124=DIRECTION('ref_axis',(1.,0.,0.));
#13125=DIRECTION('',(-1.,-1.23908819712629E-16,0.));
#13126=DIRECTION('',(1.,1.23908819712629E-16,0.));
#13127=DIRECTION('center_axis',(1.,1.23908819712629E-16,0.));
#13128=DIRECTION('ref_axis',(-1.23908819712629E-16,1.,0.));
#13129=DIRECTION('center_axis',(-1.,-1.23908819712629E-16,0.));
#13130=DIRECTION('ref_axis',(1.23908819712629E-16,-1.,0.));
#13131=DIRECTION('center_axis',(-0.866025403784436,0.,-0.500000000000005));
#13132=DIRECTION('ref_axis',(0.,1.,0.));
#13133=DIRECTION('center_axis',(0.,0.,1.));
#13134=DIRECTION('ref_axis',(1.,0.,0.));
#13135=DIRECTION('',(1.,0.,0.));
#13136=DIRECTION('',(-1.,-2.89120579329468E-17,0.));
#13137=DIRECTION('center_axis',(0.,-1.,0.));
#13138=DIRECTION('ref_axis',(0.,0.,-1.));
#13139=DIRECTION('center_axis',(-2.89120579329468E-17,1.,0.));
#13140=DIRECTION('ref_axis',(-1.,-2.89120579329468E-17,0.));
#16272=CARTESIAN_POINT('',(0.,0.,0.));
#16273=CARTESIAN_POINT('Origin',(171.5,0.,9.));
#16274=CARTESIAN_POINT('',(167.5,-4.89858719658942E-16,4.6));
#16275=CARTESIAN_POINT('Origin',(171.5,0.,4.6));
#16276=CARTESIAN_POINT('',(167.5,-4.89858719658721E-16,13.1339745962156));
#16277=CARTESIAN_POINT('',(167.5,-4.89858719658942E-16,9.));
#16278=CARTESIAN_POINT('',(169.886751345948,-3.66024982483438,9.));
#16279=CARTESIAN_POINT('Origin',(171.5,-6.00377027238687E-14,6.20577136594074));
#16280=CARTESIAN_POINT('',(169.886751345948,3.66024982483438,9.));
#16281=CARTESIAN_POINT('Origin',(171.5,0.,9.));
#16282=CARTESIAN_POINT('Origin',(171.5,-6.00377027238687E-14,6.20577136594074));
#16283=CARTESIAN_POINT('Origin',(171.5,0.,9.));
#16284=CARTESIAN_POINT('',(169.25,-2.75545529808155E-16,1.));
#16285=CARTESIAN_POINT('Origin',(171.5,0.,1.));
#16286=CARTESIAN_POINT('',(169.25,-2.75545529808155E-16,4.6));
#16287=CARTESIAN_POINT('',(169.25,-2.75545529808155E-16,9.));
#16288=CARTESIAN_POINT('Origin',(171.5,0.,4.6));
#16289=CARTESIAN_POINT('Origin',(183.5,0.,9.));
#16290=CARTESIAN_POINT('',(179.5,-4.89858719658942E-16,4.6));
#16291=CARTESIAN_POINT('Origin',(183.5,0.,4.6));
#16292=CARTESIAN_POINT('',(179.5,-4.89858719658942E-16,9.));
#16293=CARTESIAN_POINT('',(179.5,-4.89858719658942E-16,9.));
#16294=CARTESIAN_POINT('Origin',(183.5,0.,9.));
#16295=CARTESIAN_POINT('Origin',(183.5,0.,9.));
#16296=CARTESIAN_POINT('',(181.25,-2.75545529808155E-16,1.));
#16297=CARTESIAN_POINT('Origin',(183.5,0.,1.));
#16298=CARTESIAN_POINT('',(181.25,-2.75545529808155E-16,4.6));
#16299=CARTESIAN_POINT('',(181.25,-2.75545529808155E-16,9.));
#16300=CARTESIAN_POINT('Origin',(183.5,0.,4.6));
#16301=CARTESIAN_POINT('Origin',(210.,2.50000000000003,9.));
#16302=CARTESIAN_POINT('',(217.,2.50000000000003,9.));
#16303=CARTESIAN_POINT('Origin',(210.,2.50000000000003,9.));
#16304=CARTESIAN_POINT('',(217.,2.50000000000003,8.));
#16305=CARTESIAN_POINT('',(217.,2.50000000000003,9.));
#16306=CARTESIAN_POINT('Origin',(210.,2.50000000000003,8.));
#16307=CARTESIAN_POINT('Origin',(210.,2.50000000000003,8.));
#16308=CARTESIAN_POINT('',(220.,2.50000000000003,8.));
#16309=CARTESIAN_POINT('Origin',(210.,2.50000000000003,8.));
#16310=CARTESIAN_POINT('',(220.,2.50000000000003,7.));
#16311=CARTESIAN_POINT('',(220.,2.50000000000003,8.));
#16312=CARTESIAN_POINT('Origin',(210.,2.50000000000003,7.));
#16313=CARTESIAN_POINT('Origin',(210.,2.50000000000003,7.));
#16314=CARTESIAN_POINT('',(221.1,2.50000000000003,7.));
#16315=CARTESIAN_POINT('Origin',(210.,2.50000000000003,7.));
#16316=CARTESIAN_POINT('',(221.1,2.50000000000003,0.));
#16317=CARTESIAN_POINT('',(221.1,2.50000000000003,7.));
#16318=CARTESIAN_POINT('Origin',(210.,2.50000000000003,0.));
#16319=CARTESIAN_POINT('Origin',(160.,-15.,3.));
#16320=CARTESIAN_POINT('',(160.,3.94999999999999,3.));
#16321=CARTESIAN_POINT('',(190.,3.94999999999999,3.));
#16322=CARTESIAN_POINT('',(190.,3.95,3.));
#16323=CARTESIAN_POINT('',(160.,13.,3.));
#16324=CARTESIAN_POINT('',(160.,-15.,3.));
#16325=CARTESIAN_POINT('',(162.,15.,3.));
#16326=CARTESIAN_POINT('Origin',(162.,13.,3.));
#16327=CARTESIAN_POINT('',(190.,15.,3.));
#16328=CARTESIAN_POINT('',(160.,15.,3.));
#16329=CARTESIAN_POINT('',(190.,-15.,3.));
#16330=CARTESIAN_POINT('Origin',(160.,-15.,3.));
#16331=CARTESIAN_POINT('',(190.,-3.95,3.));
#16332=CARTESIAN_POINT('',(160.,-3.95,3.));
#16333=CARTESIAN_POINT('',(190.,-3.95,3.));
#16334=CARTESIAN_POINT('',(190.,-15.,3.));
#16335=CARTESIAN_POINT('',(190.,-15.,3.));
#16336=CARTESIAN_POINT('',(162.,-15.,3.));
#16337=CARTESIAN_POINT('',(160.,-15.,3.));
#16338=CARTESIAN_POINT('',(160.,-13.,3.));
#16339=CARTESIAN_POINT('Origin',(162.,-13.,3.));
#16340=CARTESIAN_POINT('',(160.,-15.,3.));
#16341=CARTESIAN_POINT('Origin',(190.,-15.,0.));
#16342=CARTESIAN_POINT('',(190.,3.95,1.));
#16343=CARTESIAN_POINT('',(190.,3.95,1.));
#16344=CARTESIAN_POINT('',(190.,15.,0.));
#16345=CARTESIAN_POINT('',(190.,15.,0.));
#16346=CARTESIAN_POINT('',(190.,-15.,0.));
#16347=CARTESIAN_POINT('',(190.,-15.,0.));
#16348=CARTESIAN_POINT('',(190.,-15.,0.));
#16349=CARTESIAN_POINT('',(190.,-3.95,1.));
#16350=CARTESIAN_POINT('',(190.,-3.95,1.));
#16351=CARTESIAN_POINT('',(190.,-3.95,1.));
#16352=CARTESIAN_POINT('Origin',(13.1197502427733,-56.2532019429921,9.));
#16353=CARTESIAN_POINT('',(212.839139451054,-9.67330222977594,0.));
#16354=CARTESIAN_POINT('',(13.1197502427733,-56.2532019429921,0.));
#16355=CARTESIAN_POINT('',(212.839139451054,-9.67330222977594,9.));
#16356=CARTESIAN_POINT('',(212.839139451054,-9.67330222977594,9.));
#16357=CARTESIAN_POINT('',(190.,-15.,9.));
#16358=CARTESIAN_POINT('',(13.1197502427733,-56.2532019429921,9.));
#16359=CARTESIAN_POINT('',(190.,-15.,9.));
#16360=CARTESIAN_POINT('Origin',(210.,2.50000000000003,9.));
#16361=CARTESIAN_POINT('',(210.,15.,0.));
#16362=CARTESIAN_POINT('Origin',(210.,2.50000000000003,0.));
#16363=CARTESIAN_POINT('',(210.,15.,9.));
#16364=CARTESIAN_POINT('',(210.,15.,9.));
#16365=CARTESIAN_POINT('Origin',(210.,2.50000000000003,9.));
#16366=CARTESIAN_POINT('Origin',(0.,15.,9.));
#16367=CARTESIAN_POINT('',(162.,15.,9.));
#16368=CARTESIAN_POINT('',(162.,15.,9.));
#16369=CARTESIAN_POINT('',(0.,15.,9.));
#16370=CARTESIAN_POINT('',(0.,15.,0.));
#16371=CARTESIAN_POINT('Origin',(160.,0.,9.));
#16372=CARTESIAN_POINT('',(160.,13.,9.));
#16373=CARTESIAN_POINT('',(160.,13.,0.));
#16374=CARTESIAN_POINT('',(160.,3.95,1.));
#16375=CARTESIAN_POINT('',(160.,3.95,1.));
#16376=CARTESIAN_POINT('',(160.,-3.95,1.));
#16377=CARTESIAN_POINT('',(160.,-3.95,1.));
#16378=CARTESIAN_POINT('',(160.,-3.95,1.));
#16379=CARTESIAN_POINT('',(160.,-13.,9.));
#16380=CARTESIAN_POINT('',(160.,-13.,9.));
#16381=CARTESIAN_POINT('',(160.,-7.50000000000002,9.));
#16382=CARTESIAN_POINT('',(160.,0.,9.));
#16383=CARTESIAN_POINT('',(160.,-7.50000000000003,15.));
#16384=CARTESIAN_POINT('',(160.,-7.50000000000003,19.));
#16385=CARTESIAN_POINT('',(160.,-3.50000000000003,19.));
#16386=CARTESIAN_POINT('Origin',(160.,-3.50000000000003,15.));
#16387=CARTESIAN_POINT('',(160.,3.49999999999997,19.));
#16388=CARTESIAN_POINT('',(160.,-7.50000000000003,19.));
#16389=CARTESIAN_POINT('',(160.,7.49999999999997,15.));
#16390=CARTESIAN_POINT('Origin',(160.,3.49999999999997,15.));
#16391=CARTESIAN_POINT('',(160.,7.49999999999998,9.));
#16392=CARTESIAN_POINT('',(160.,7.49999999999997,19.));
#16393=CARTESIAN_POINT('',(160.,0.,9.));
#16394=CARTESIAN_POINT('Origin',(1.73472347597681E-15,-15.,9.));
#16395=CARTESIAN_POINT('',(162.,-15.,9.));
#16396=CARTESIAN_POINT('',(162.,-15.,9.));
#16397=CARTESIAN_POINT('',(1.73472347597681E-15,-15.,9.));
#16398=CARTESIAN_POINT('Origin',(0.,0.,9.));
#16399=CARTESIAN_POINT('',(169.886751345948,7.49999999999998,9.));
#16400=CARTESIAN_POINT('',(167.,7.49999999999998,9.));
#16401=CARTESIAN_POINT('',(169.886751345948,0.,9.));
#16402=CARTESIAN_POINT('',(169.886751345948,-7.50000000000002,9.));
#16403=CARTESIAN_POINT('',(169.886751345948,0.,9.));
#16404=CARTESIAN_POINT('',(167.,-7.50000000000002,9.));
#16405=CARTESIAN_POINT('Origin',(162.,-13.,9.));
#16406=CARTESIAN_POINT('Origin',(162.,13.,9.));
#16407=CARTESIAN_POINT('Origin',(0.,0.,0.));
#16408=CARTESIAN_POINT('Origin',(210.,2.50000000000003,7.));
#16409=CARTESIAN_POINT('Origin',(210.,2.50000000000003,8.));
#16410=CARTESIAN_POINT('Origin',(162.,-13.,9.));
#16411=CARTESIAN_POINT('Origin',(162.,13.,9.));
#16412=CARTESIAN_POINT('Origin',(185.75,0.,4.6));
#16413=CARTESIAN_POINT('Origin',(173.75,0.,4.6));
#16414=CARTESIAN_POINT('Origin',(167.,-7.50000000000002,19.));
#16415=CARTESIAN_POINT('',(167.,-7.50000000000002,15.));
#16416=CARTESIAN_POINT('',(167.,-7.50000000000002,14.));
#16417=CARTESIAN_POINT('',(167.,-7.50000000000002,19.));
#16418=CARTESIAN_POINT('',(160.,-7.50000000000003,15.));
#16419=CARTESIAN_POINT('',(164.834936490539,-7.50000000000002,17.75));
#16420=CARTESIAN_POINT('Origin',(167.,-7.50000000000002,19.));
#16421=CARTESIAN_POINT('',(167.,7.49999999999998,14.));
#16422=CARTESIAN_POINT('',(167.,-7.50000000000002,14.));
#16423=CARTESIAN_POINT('',(167.,7.49999999999998,15.));
#16424=CARTESIAN_POINT('',(167.,7.49999999999998,19.));
#16425=CARTESIAN_POINT('',(167.,3.49999999999998,19.));
#16426=CARTESIAN_POINT('Origin',(167.,3.49999999999998,15.));
#16427=CARTESIAN_POINT('',(167.,-3.50000000000002,19.));
#16428=CARTESIAN_POINT('',(167.,-7.50000000000002,19.));
#16429=CARTESIAN_POINT('Origin',(167.,-3.50000000000002,15.));
#16430=CARTESIAN_POINT('Origin',(167.,7.49999999999998,19.));
#16431=CARTESIAN_POINT('',(167.,7.49999999999998,15.));
#16432=CARTESIAN_POINT('',(164.834936490539,7.49999999999998,17.75));
#16433=CARTESIAN_POINT('Origin',(0.,0.,19.));
#16434=CARTESIAN_POINT('',(160.,3.49999999999997,19.));
#16435=CARTESIAN_POINT('',(167.,-3.50000000000002,19.));
#16436=CARTESIAN_POINT('Origin',(-4.33680868994196E-16,3.49999999999995,
15.));
#16437=CARTESIAN_POINT('Origin',(4.33680868994207E-16,-3.50000000000005,
15.));
#16438=CARTESIAN_POINT('Origin',(167.,-7.50000000000002,14.));
#16439=CARTESIAN_POINT('Origin',(0.,0.,1.));
#16440=CARTESIAN_POINT('',(190.,3.95,1.));
#16441=CARTESIAN_POINT('',(190.,-3.95,1.));
#16442=CARTESIAN_POINT('Origin',(190.,3.95,1.));
#16443=CARTESIAN_POINT('Origin',(190.,-3.95,1.));
#18836=UNCERTAINTY_MEASURE_WITH_UNIT(LENGTH_MEASURE(0.01),#18868,
'DISTANCE_ACCURACY_VALUE',
'Maximum model space distance between geometric entities at asserted c
onnectivities');
#18849=UNCERTAINTY_MEASURE_WITH_UNIT(LENGTH_MEASURE(0.01),#18868,
'DISTANCE_ACCURACY_VALUE',
'Maximum model space distance between geometric entities at asserted c
onnectivities');
#18854=(
GEOMETRIC_REPRESENTATION_CONTEXT(3)
GLOBAL_UNCERTAINTY_ASSIGNED_CONTEXT((#18836))
GLOBAL_UNIT_ASSIGNED_CONTEXT((#18868,#18870,#18871))
REPRESENTATION_CONTEXT('','3D')
);
#18867=(
GEOMETRIC_REPRESENTATION_CONTEXT(3)
GLOBAL_UNCERTAINTY_ASSIGNED_CONTEXT((#18849))
GLOBAL_UNIT_ASSIGNED_CONTEXT((#18868,#18870,#18871))
REPRESENTATION_CONTEXT('','3D')
);
#18868=(
LENGTH_UNIT()
NAMED_UNIT(*)
SI_UNIT(.MILLI.,.METRE.)
);
#18870=(
NAMED_UNIT(*)
PLANE_ANGLE_UNIT()
SI_UNIT($,.RADIAN.)
);
#18871=(
NAMED_UNIT(*)
SI_UNIT($,.STERADIAN.)
SOLID_ANGLE_UNIT()
);
#18876=SHAPE_DEFINITION_REPRESENTATION(#18893,#18938);
#18893=PRODUCT_DEFINITION_SHAPE('',$,#18956);
#18938=SHAPE_REPRESENTATION('',(#11366),#18854);
#18951=PRODUCT_DEFINITION_CONTEXT('part definition',#19004,'design');
#18956=PRODUCT_DEFINITION('Idler End Bracket 2','Idler End Bracket 2',#18973,
#18951);
#18973=PRODUCT_DEFINITION_FORMATION('',$,#19010);
#19004=APPLICATION_CONTEXT(
'Core Data for Automotive Mechanical Design Process');
#19005=PRODUCT_CONTEXT('part definition',#19004,'mechanical');
#19010=PRODUCT('Idler End Bracket 2','Idler End Bracket 2',$,(#19005));
#19025=PRESENTATION_STYLE_ASSIGNMENT((#19031));
#19031=SURFACE_STYLE_USAGE(.BOTH.,#19037);
#19037=SURFACE_SIDE_STYLE('',(#19043));
#19043=SURFACE_STYLE_FILL_AREA(#19049);
#19049=FILL_AREA_STYLE('Opaque(97,158,199)',(#19055));
#19055=FILL_AREA_STYLE_COLOUR('Opaque(97,158,199)',#19061);
#19061=COLOUR_RGB('Opaque(97,158,199)',0.380392156862745,0.619607843137255,
0.780392156862745);
ENDSEC;
END-ISO-10303-21;
